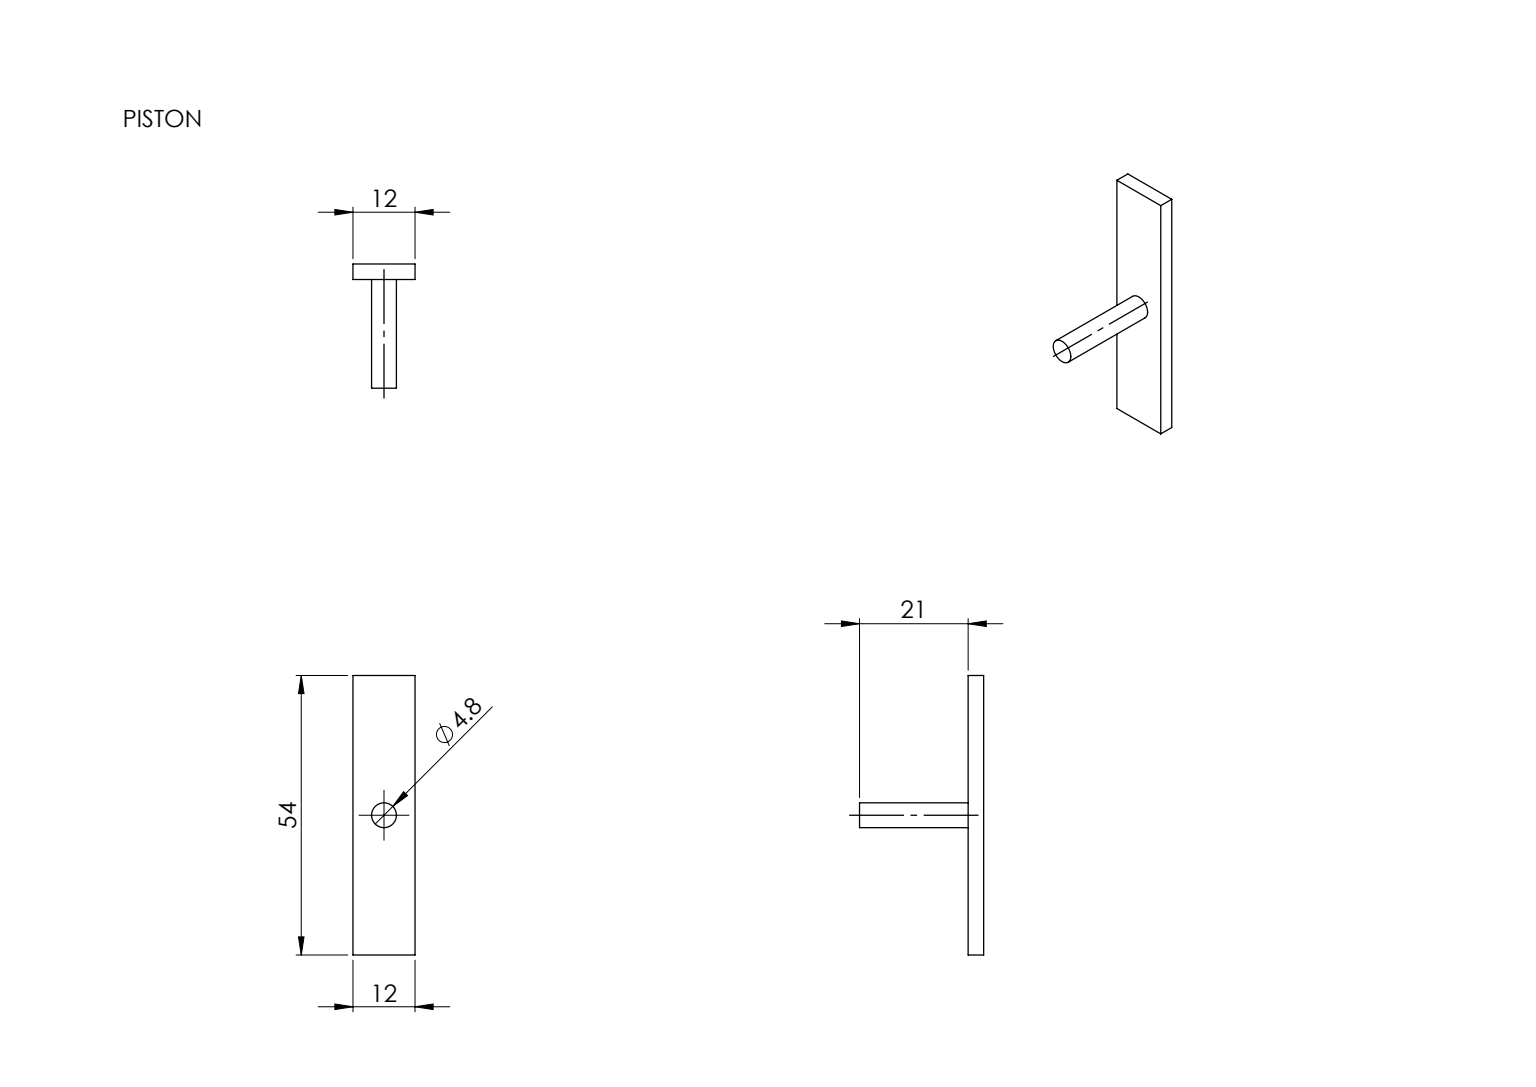
ISO-10303-21;
HEADER;
FILE_DESCRIPTION (('STEP AP214'),
    '1' );
FILE_NAME ('piston.step',
    '2026-10-03T18:28:46',
    ( '' ),
    ( '' ),
    'SwSTEP 2.0',
    'SolidWorks 2026',
    '' );
FILE_SCHEMA (( 'AUTOMOTIVE_DESIGN' ));
ENDSEC;

DATA;
#3=DIRECTION ( 'NONE',  ( -1.000000000000000000, 0.000000000000000000, 0.000000000000000000 ) ) ;
#13=SHAPE_REPRESENTATION ( 'piston', ( #2101 ), #6502 ) ;
#16=PRODUCT_CONTEXT ( 'NONE', #527, 'mechanical' ) ;
#52=ORIENTED_EDGE ( 'NONE', *, *, #338, .F. ) ;
#110=CARTESIAN_POINT ( 'NONE',  ( 5.999999999999999112, -27.00000000000000711, -14.00000000000000178 ) ) ;
#132=LINE ( 'NONE', #5884, #6142 ) ;
#157=CARTESIAN_POINT ( 'NONE',  ( 0.000000000000000000, 0.000000000000000000, 6.999999999999999112 ) ) ;
#184=DIRECTION ( 'NONE',  ( -0.000000000000000000, -0.000000000000000000, -1.000000000000000000 ) ) ;
#232=LINE ( 'NONE', #7430, #6006 ) ;
#246=LINE ( 'NONE', #6800, #847 ) ;
#249=DIRECTION ( 'NONE',  ( -1.000000000000000000, 0.000000000000000000, 0.000000000000000000 ) ) ;
#338=EDGE_CURVE ( 'NONE', #7188, #9680, #5880, .T. ) ;
#349=DIRECTION ( 'NONE',  ( -0.000000000000000000, -1.000000000000000000, -0.000000000000000000 ) ) ;
#383=DIRECTION ( 'NONE',  ( 0.000000000000000000, 0.000000000000000000, 1.000000000000000000 ) ) ;
#496=PRODUCT_DEFINITION ( 'UNKNOWN', '', #10431, #818 ) ;
#527=APPLICATION_CONTEXT ( 'automotive_design' ) ;
#544=ORIENTED_EDGE ( 'NONE', *, *, #10139, .T. ) ;
#558=AXIS2_PLACEMENT_3D ( 'NONE', #2527, #5797, #5015 ) ;
#728=SURFACE_STYLE_USAGE ( .BOTH. , #9540 ) ;
#770=ORIENTED_EDGE ( 'NONE', *, *, #4732, .T. ) ;
#776=ORIENTED_EDGE ( 'NONE', *, *, #9858, .T. ) ;
#779=ORIENTED_EDGE ( 'NONE', *, *, #1512, .F. ) ;
#800=CARTESIAN_POINT ( 'NONE',  ( 2.399999999999999911, 2.939152317953647106E-16, 6.999999999999999112 ) ) ;
#818=PRODUCT_DEFINITION_CONTEXT ( 'detailed design', #5599, 'design' ) ;
#847=VECTOR ( 'NONE', #349, 1000.000000000000000 ) ;
#850=FACE_OUTER_BOUND ( 'NONE', #7920, .T. ) ;
#852=FACE_OUTER_BOUND ( 'NONE', #4523, .T. ) ;
#862=DIRECTION ( 'NONE',  ( 1.000000000000000000, 0.000000000000000000, 0.000000000000000000 ) ) ;
#932=AXIS2_PLACEMENT_3D ( 'NONE', #1647, #10350, #3 ) ;
#956=LINE ( 'NONE', #800, #10182 ) ;
#982=PRESENTATION_STYLE_ASSIGNMENT (( #8411 ) ) ;
#1012=CARTESIAN_POINT ( 'NONE',  ( 0.000000000000000000, 0.000000000000000000, 6.999999999999999112 ) ) ;
#1038=FILL_AREA_STYLE ('',( #3422 ) ) ;
#1126=DIRECTION ( 'NONE',  ( -0.000000000000000000, -0.000000000000000000, -1.000000000000000000 ) ) ;
#1159=DIRECTION ( 'NONE',  ( 0.000000000000000000, 1.000000000000000000, 0.000000000000000000 ) ) ;
#1267=CARTESIAN_POINT ( 'NONE',  ( 5.999999999999999112, 26.99999999999999289, -14.00000000000000178 ) ) ;
#1289=CARTESIAN_POINT ( 'NONE',  ( 5.999999999999999112, 26.99999999999999289, -17.00000000000000000 ) ) ;
#1300=LINE ( 'NONE', #5952, #9319 ) ;
#1316=DIRECTION ( 'NONE',  ( -0.000000000000000000, -0.000000000000000000, -1.000000000000000000 ) ) ;
#1319=CARTESIAN_POINT ( 'NONE',  ( 5.999999999999999112, 26.99999999999999289, -14.00000000000000178 ) ) ;
#1475=CARTESIAN_POINT ( 'NONE',  ( -5.999999999999999112, -27.00000000000000711, -14.00000000000000178 ) ) ;
#1483=ORIENTED_EDGE ( 'NONE', *, *, #8967, .F. ) ;
#1486=ADVANCED_FACE ( 'NONE', ( #5139 ), #9931, .T. ) ;
#1512=EDGE_CURVE ( 'NONE', #9680, #4528, #7119, .T. ) ;
#1647=CARTESIAN_POINT ( 'NONE',  ( 0.000000000000000000, 0.000000000000000000, 6.999999999999999112 ) ) ;
#1677=CARTESIAN_POINT ( 'NONE',  ( 0.000000000000000000, 0.000000000000000000, -14.00000000000000178 ) ) ;
#1697=VERTEX_POINT ( 'NONE', #1319 ) ;
#1711=LINE ( 'NONE', #1866, #9206 ) ;
#1794=EDGE_LOOP ( 'NONE', ( #779, #4050 ) ) ;
#1812=DIRECTION ( 'NONE',  ( 0.000000000000000000, 0.000000000000000000, 1.000000000000000000 ) ) ;
#1814=LINE ( 'NONE', #3454, #9036 ) ;
#1866=CARTESIAN_POINT ( 'NONE',  ( -5.999999999999999112, 26.99999999999999289, -14.00000000000000178 ) ) ;
#1945=DIRECTION ( 'NONE',  ( 0.000000000000000000, 1.000000000000000000, -0.000000000000000000 ) ) ;
#1968=AXIS2_PLACEMENT_3D ( 'NONE', #4462, #8603, #7710 ) ;
#2042=SURFACE_SIDE_STYLE ('',( #6743 ) ) ;
#2050=PLANE ( 'NONE',  #6514 ) ;
#2063=ORIENTED_EDGE ( 'NONE', *, *, #9661, .F. ) ;
#2101=AXIS2_PLACEMENT_3D ( 'NONE', #7090, #5610, #4547 ) ;
#2278=EDGE_CURVE ( 'NONE', #7564, #10476, #6459, .T. ) ;
#2305=EDGE_CURVE ( 'NONE', #8379, #4528, #956, .T. ) ;
#2325=FACE_OUTER_BOUND ( 'NONE', #3648, .T. ) ;
#2338=ADVANCED_FACE ( 'NONE', ( #850 ), #4028, .F. ) ;
#2527=CARTESIAN_POINT ( 'NONE',  ( 0.000000000000000000, 0.000000000000000000, 6.999999999999999112 ) ) ;
#2583=ORIENTED_EDGE ( 'NONE', *, *, #3437, .T. ) ;
#2597=VECTOR ( 'NONE', #4595, 1000.000000000000000 ) ;
#2620=VECTOR ( 'NONE', #1316, 1000.000000000000000 ) ;
#2680=FACE_OUTER_BOUND ( 'NONE', #7404, .T. ) ;
#2743=ORIENTED_EDGE ( 'NONE', *, *, #3577, .T. ) ;
#2758=ORIENTED_EDGE ( 'NONE', *, *, #9103, .F. ) ;
#2818=AXIS2_PLACEMENT_3D ( 'NONE', #6404, #8911, #6513 ) ;
#2874=ORIENTED_EDGE ( 'NONE', *, *, #9103, .T. ) ;
#2957=SHAPE_REPRESENTATION_RELATIONSHIP ( 'NONE' , 'NONE' ,  #13, #2960 ) ;
#2960=ADVANCED_BREP_SHAPE_REPRESENTATION ( '', ( #4712, #2101 ), #6502 ) ;
#2964=DIRECTION ( 'NONE',  ( 0.000000000000000000, 0.000000000000000000, -1.000000000000000000 ) ) ;
#2976=CARTESIAN_POINT ( 'NONE',  ( -2.399999999999999911, 0.000000000000000000, 6.999999999999999112 ) ) ;
#3047=( GEOMETRIC_REPRESENTATION_CONTEXT ( 3 ) GLOBAL_UNCERTAINTY_ASSIGNED_CONTEXT ( ( #6318 ) ) GLOBAL_UNIT_ASSIGNED_CONTEXT ( ( #3624, #9954, #10058 ) ) REPRESENTATION_CONTEXT ( 'NONE', 'WORKASPACE' ) );
#3049=VERTEX_POINT ( 'NONE', #1289 ) ;
#3068=ADVANCED_FACE ( 'NONE', ( #3618 ), #6847, .F. ) ;
#3069=PLANE ( 'NONE',  #10326 ) ;
#3098=VECTOR ( 'NONE', #1159, 1000.000000000000000 ) ;
#3214=ORIENTED_EDGE ( 'NONE', *, *, #8056, .T. ) ;
#3218=AXIS2_PLACEMENT_3D ( 'NONE', #1677, #8203, #6490 ) ;
#3337=DIRECTION ( 'NONE',  ( 1.000000000000000000, -0.000000000000000000, -0.000000000000000000 ) ) ;
#3366=FACE_BOUND ( 'NONE', #1794, .T. ) ;
#3383=ORIENTED_EDGE ( 'NONE', *, *, #9858, .F. ) ;
#3422=FILL_AREA_STYLE_COLOUR ( '', #7101 ) ;
#3437=EDGE_CURVE ( 'NONE', #5860, #7564, #232, .T. ) ;
#3441=DIRECTION ( 'NONE',  ( 0.000000000000000000, 0.000000000000000000, 1.000000000000000000 ) ) ;
#3454=CARTESIAN_POINT ( 'NONE',  ( 5.999999999999999112, -27.00000000000000711, -17.00000000000000000 ) ) ;
#3501=ORIENTED_EDGE ( 'NONE', *, *, #10055, .T. ) ;
#3577=EDGE_CURVE ( 'NONE', #4528, #9680, #4318, .T. ) ;
#3592=( NAMED_UNIT ( * ) SI_UNIT ( $, .STERADIAN. ) SOLID_ANGLE_UNIT ( ) );
#3618=FACE_OUTER_BOUND ( 'NONE', #8196, .T. ) ;
#3624=( LENGTH_UNIT ( ) NAMED_UNIT ( * ) SI_UNIT ( .MILLI., .METRE. ) );
#3648=EDGE_LOOP ( 'NONE', ( #2583, #3383, #4167, #544 ) ) ;
#3662=CARTESIAN_POINT ( 'NONE',  ( 0.000000000000000000, 0.000000000000000000, -14.00000000000000178 ) ) ;
#3724=CARTESIAN_POINT ( 'NONE',  ( -5.999999999999999112, 26.99999999999999289, -14.00000000000000178 ) ) ;
#3725=ORIENTED_EDGE ( 'NONE', *, *, #5954, .T. ) ;
#3745=PRESENTATION_STYLE_ASSIGNMENT (( #728 ) ) ;
#3851=SURFACE_STYLE_FILL_AREA ( #6975 ) ;
#3863=CYLINDRICAL_SURFACE ( 'NONE', #932, 2.399999999999999911 ) ;
#3877=FACE_OUTER_BOUND ( 'NONE', #4533, .T. ) ;
#3891=ADVANCED_FACE ( 'NONE', ( #852 ), #4030, .F. ) ;
#3960=( NAMED_UNIT ( * ) PLANE_ANGLE_UNIT ( ) SI_UNIT ( $, .RADIAN. ) );
#3974=STYLED_ITEM ( 'NONE', ( #3745 ), #2960 ) ;
#4028=PLANE ( 'NONE',  #8996 ) ;
#4030=PLANE ( 'NONE',  #2818 ) ;
#4050=ORIENTED_EDGE ( 'NONE', *, *, #3577, .F. ) ;
#4081=CARTESIAN_POINT ( 'NONE',  ( 5.999999999999999112, 26.99999999999999289, -14.00000000000000178 ) ) ;
#4167=ORIENTED_EDGE ( 'NONE', *, *, #4732, .F. ) ;
#4242=DIRECTION ( 'NONE',  ( 0.000000000000000000, 1.000000000000000000, 0.000000000000000000 ) ) ;
#4291=ADVANCED_FACE ( 'NONE', ( #2325 ), #3069, .F. ) ;
#4292=DIRECTION ( 'NONE',  ( -0.000000000000000000, -0.000000000000000000, -1.000000000000000000 ) ) ;
#4304=MECHANICAL_DESIGN_GEOMETRIC_PRESENTATION_REPRESENTATION('',(#3974),#7361);
#4318=CIRCLE ( 'NONE', #5674, 2.399999999999999911 ) ;
#4340=DIRECTION ( 'NONE',  ( 1.000000000000000000, 0.000000000000000000, 0.000000000000000000 ) ) ;
#4385=CLOSED_SHELL ( 'NONE', ( #5658, #3891, #2338, #4291, #6602, #4600, #3068, #1486, #9647 ) ) ;
#4391=CARTESIAN_POINT ( 'NONE',  ( 0.000000000000000000, 0.000000000000000000, -14.00000000000000178 ) ) ;
#4462=CARTESIAN_POINT ( 'NONE',  ( 0.000000000000000000, 0.000000000000000000, -17.00000000000000000 ) ) ;
#4523=EDGE_LOOP ( 'NONE', ( #3501, #2758, #1483, #3725 ) ) ;
#4528=VERTEX_POINT ( 'NONE', #7348 ) ;
#4533=EDGE_LOOP ( 'NONE', ( #6599, #5263, #6529, #776 ) ) ;
#4547=DIRECTION ( 'NONE',  ( 1.000000000000000000, 0.000000000000000000, 0.000000000000000000 ) ) ;
#4568=VERTEX_POINT ( 'NONE', #10495 ) ;
#4595=DIRECTION ( 'NONE',  ( -1.000000000000000000, 0.000000000000000000, 0.000000000000000000 ) ) ;
#4600=ADVANCED_FACE ( 'NONE', ( #3366, #9047 ), #4957, .T. ) ;
#4705=FACE_OUTER_BOUND ( 'NONE', #5856, .T. ) ;
#4712=MANIFOLD_SOLID_BREP ( 'Boss-Extrude2', #4385 ) ;
#4732=EDGE_CURVE ( 'NONE', #8579, #4568, #246, .T. ) ;
#4746=AXIS2_PLACEMENT_3D ( 'NONE', #4391, #1812, #4340 ) ;
#4767=ORIENTED_EDGE ( 'NONE', *, *, #8967, .T. ) ;
#4821=DIRECTION ( 'NONE',  ( 0.000000000000000000, -0.000000000000000000, -1.000000000000000000 ) ) ;
#4882=DIRECTION ( 'NONE',  ( 0.000000000000000000, 0.000000000000000000, 1.000000000000000000 ) ) ;
#4924=AXIS2_PLACEMENT_3D ( 'NONE', #5873, #5824, #8339 ) ;
#4957=PLANE ( 'NONE',  #3218 ) ;
#5015=DIRECTION ( 'NONE',  ( 1.000000000000000000, 0.000000000000000000, -0.000000000000000000 ) ) ;
#5029=DIRECTION ( 'NONE',  ( -0.000000000000000000, -0.000000000000000000, -1.000000000000000000 ) ) ;
#5078=CARTESIAN_POINT ( 'NONE',  ( -5.999999999999999112, 26.99999999999999289, -17.00000000000000000 ) ) ;
#5119=ORIENTED_EDGE ( 'NONE', *, *, #10139, .F. ) ;
#5139=FACE_OUTER_BOUND ( 'NONE', #9744, .T. ) ;
#5167=ORIENTED_EDGE ( 'NONE', *, *, #338, .T. ) ;
#5230=FILL_AREA_STYLE_COLOUR ( '', #8549 ) ;
#5232=ORIENTED_EDGE ( 'NONE', *, *, #2305, .T. ) ;
#5263=ORIENTED_EDGE ( 'NONE', *, *, #5954, .F. ) ;
#5406=MECHANICAL_DESIGN_GEOMETRIC_PRESENTATION_REPRESENTATION('',(#6249),#3047);
#5427=VECTOR ( 'NONE', #3337, 1000.000000000000000 ) ;
#5599=APPLICATION_CONTEXT ( 'automotive_design' ) ;
#5610=DIRECTION ( 'NONE',  ( 0.000000000000000000, 0.000000000000000000, 1.000000000000000000 ) ) ;
#5658=ADVANCED_FACE ( 'NONE', ( #4705 ), #3863, .T. ) ;
#5674=AXIS2_PLACEMENT_3D ( 'NONE', #3662, #383, #10143 ) ;
#5765=CARTESIAN_POINT ( 'NONE',  ( 5.999999999999999112, -27.00000000000000711, -17.00000000000000000 ) ) ;
#5797=DIRECTION ( 'NONE',  ( 0.000000000000000000, 0.000000000000000000, 1.000000000000000000 ) ) ;
#5824=DIRECTION ( 'NONE',  ( -0.000000000000000000, -0.000000000000000000, -1.000000000000000000 ) ) ;
#5850=CARTESIAN_POINT ( 'NONE',  ( 5.999999999999999112, 26.99999999999999289, -17.00000000000000000 ) ) ;
#5856=EDGE_LOOP ( 'NONE', ( #9307, #5232, #2743, #52 ) ) ;
#5860=VERTEX_POINT ( 'NONE', #5078 ) ;
#5870=EDGE_CURVE ( 'NONE', #8379, #7188, #5987, .T. ) ;
#5873=CARTESIAN_POINT ( 'NONE',  ( 0.000000000000000000, 0.000000000000000000, 6.999999999999999112 ) ) ;
#5880=LINE ( 'NONE', #6034, #10471 ) ;
#5884=CARTESIAN_POINT ( 'NONE',  ( -5.999999999999999112, -27.00000000000000711, -14.00000000000000178 ) ) ;
#5897=CARTESIAN_POINT ( 'NONE',  ( -2.399999999999999911, 0.000000000000000000, -14.00000000000000178 ) ) ;
#5916=LINE ( 'NONE', #110, #8219 ) ;
#5950=ORIENTED_EDGE ( 'NONE', *, *, #1512, .T. ) ;
#5951=DIRECTION ( 'NONE',  ( 0.000000000000000000, 0.000000000000000000, 1.000000000000000000 ) ) ;
#5952=CARTESIAN_POINT ( 'NONE',  ( 5.999999999999999112, -27.00000000000000711, -14.00000000000000178 ) ) ;
#5954=EDGE_CURVE ( 'NONE', #9536, #10476, #5916, .T. ) ;
#5987=CIRCLE ( 'NONE', #10085, 2.399999999999999911 ) ;
#6006=VECTOR ( 'NONE', #8185, 1000.000000000000000 ) ;
#6034=CARTESIAN_POINT ( 'NONE',  ( -2.399999999999999911, 0.000000000000000000, 6.999999999999999112 ) ) ;
#6125=( LENGTH_UNIT ( ) NAMED_UNIT ( * ) SI_UNIT ( .MILLI., .METRE. ) );
#6142=VECTOR ( 'NONE', #184, 1000.000000000000000 ) ;
#6233=CARTESIAN_POINT ( 'NONE',  ( 5.999999999999999112, 26.99999999999999289, -14.00000000000000178 ) ) ;
#6249=STYLED_ITEM ( 'NONE', ( #982 ), #4712 ) ;
#6309=CARTESIAN_POINT ( 'NONE',  ( 5.999999999999999112, -27.00000000000000711, -14.00000000000000178 ) ) ;
#6318=UNCERTAINTY_MEASURE_WITH_UNIT (LENGTH_MEASURE( 1.000000000000000082E-05 ), #3624, 'distance_accuracy_value', 'NONE');
#6331=ORIENTED_EDGE ( 'NONE', *, *, #3437, .F. ) ;
#6344=DIRECTION ( 'NONE',  ( 1.000000000000000000, 0.000000000000000000, 0.000000000000000000 ) ) ;
#6347=ORIENTED_EDGE ( 'NONE', *, *, #10055, .F. ) ;
#6404=CARTESIAN_POINT ( 'NONE',  ( 5.999999999999999112, -27.00000000000000711, -14.00000000000000178 ) ) ;
#6459=LINE ( 'NONE', #5765, #5427 ) ;
#6474=PRODUCT_DEFINITION_SHAPE ( 'NONE', 'NONE',  #496 ) ;
#6490=DIRECTION ( 'NONE',  ( 1.000000000000000000, 0.000000000000000000, -0.000000000000000000 ) ) ;
#6502=( GEOMETRIC_REPRESENTATION_CONTEXT ( 3 ) GLOBAL_UNCERTAINTY_ASSIGNED_CONTEXT ( ( #7923 ) ) GLOBAL_UNIT_ASSIGNED_CONTEXT ( ( #6763, #7623, #3592 ) ) REPRESENTATION_CONTEXT ( 'NONE', 'WORKASPACE' ) );
#6509=ORIENTED_EDGE ( 'NONE', *, *, #9021, .T. ) ;
#6513=DIRECTION ( 'NONE',  ( 0.000000000000000000, 0.000000000000000000, 1.000000000000000000 ) ) ;
#6514=AXIS2_PLACEMENT_3D ( 'NONE', #6309, #1945, #5951 ) ;
#6529=ORIENTED_EDGE ( 'NONE', *, *, #8056, .F. ) ;
#6547=PLANE ( 'NONE',  #558 ) ;
#6599=ORIENTED_EDGE ( 'NONE', *, *, #2278, .T. ) ;
#6602=ADVANCED_FACE ( 'NONE', ( #3877 ), #2050, .F. ) ;
#6672=ORIENTED_EDGE ( 'NONE', *, *, #10200, .T. ) ;
#6743=SURFACE_STYLE_FILL_AREA ( #1038 ) ;
#6763=( LENGTH_UNIT ( ) NAMED_UNIT ( * ) SI_UNIT ( .MILLI., .METRE. ) );
#6800=CARTESIAN_POINT ( 'NONE',  ( -5.999999999999999112, -27.00000000000000711, -14.00000000000000178 ) ) ;
#6817=VECTOR ( 'NONE', #249, 1000.000000000000000 ) ;
#6847=PLANE ( 'NONE',  #1968 ) ;
#6975=FILL_AREA_STYLE ('',( #5230 ) ) ;
#6998=CIRCLE ( 'NONE', #9899, 2.399999999999999911 ) ;
#7030=CARTESIAN_POINT ( 'NONE',  ( -5.999999999999999112, -27.00000000000000711, -17.00000000000000000 ) ) ;
#7090=CARTESIAN_POINT ( 'NONE',  ( 0.000000000000000000, 0.000000000000000000, 0.000000000000000000 ) ) ;
#7101=COLOUR_RGB ( '', 0.72549020, 0.75294118, 0.79215686) ;
#7119=CIRCLE ( 'NONE', #4746, 2.399999999999999911 ) ;
#7184=ORIENTED_EDGE ( 'NONE', *, *, #9661, .T. ) ;
#7188=VERTEX_POINT ( 'NONE', #2976 ) ;
#7348=CARTESIAN_POINT ( 'NONE',  ( 2.399999999999999911, 2.939152317953647106E-16, -14.00000000000000178 ) ) ;
#7361=( GEOMETRIC_REPRESENTATION_CONTEXT ( 3 ) GLOBAL_UNCERTAINTY_ASSIGNED_CONTEXT ( ( #10125 ) ) GLOBAL_UNIT_ASSIGNED_CONTEXT ( ( #6125, #3960, #9483 ) ) REPRESENTATION_CONTEXT ( 'NONE', 'WORKASPACE' ) );
#7404=EDGE_LOOP ( 'NONE', ( #6672, #9721 ) ) ;
#7430=CARTESIAN_POINT ( 'NONE',  ( -5.999999999999999112, -27.00000000000000711, -17.00000000000000000 ) ) ;
#7564=VERTEX_POINT ( 'NONE', #7030 ) ;
#7623=( NAMED_UNIT ( * ) PLANE_ANGLE_UNIT ( ) SI_UNIT ( $, .RADIAN. ) );
#7710=DIRECTION ( 'NONE',  ( 1.000000000000000000, 0.000000000000000000, -0.000000000000000000 ) ) ;
#7827=DIRECTION ( 'NONE',  ( 1.000000000000000000, -0.000000000000000000, -0.000000000000000000 ) ) ;
#7838=LINE ( 'NONE', #1267, #2597 ) ;
#7920=EDGE_LOOP ( 'NONE', ( #7184, #5119, #8733, #2874 ) ) ;
#7923=UNCERTAINTY_MEASURE_WITH_UNIT (LENGTH_MEASURE( 1.000000000000000082E-05 ), #6763, 'distance_accuracy_value', 'NONE');
#8025=SHAPE_DEFINITION_REPRESENTATION ( #6474, #13 ) ;
#8056=EDGE_CURVE ( 'NONE', #4568, #9536, #1300, .T. ) ;
#8136=LINE ( 'NONE', #9224, #3098 ) ;
#8185=DIRECTION ( 'NONE',  ( -0.000000000000000000, -1.000000000000000000, -0.000000000000000000 ) ) ;
#8196=EDGE_LOOP ( 'NONE', ( #6347, #9272, #6331, #2063 ) ) ;
#8203=DIRECTION ( 'NONE',  ( 0.000000000000000000, -0.000000000000000000, 1.000000000000000000 ) ) ;
#8212=EDGE_LOOP ( 'NONE', ( #4767, #6509, #770, #3214 ) ) ;
#8219=VECTOR ( 'NONE', #5029, 1000.000000000000000 ) ;
#8339=DIRECTION ( 'NONE',  ( -1.000000000000000000, 0.000000000000000000, 0.000000000000000000 ) ) ;
#8379=VERTEX_POINT ( 'NONE', #8989 ) ;
#8411=SURFACE_STYLE_USAGE ( .BOTH. , #2042 ) ;
#8549=COLOUR_RGB ( '', 0.72549020, 0.75294118, 0.79215686) ;
#8579=VERTEX_POINT ( 'NONE', #3724 ) ;
#8603=DIRECTION ( 'NONE',  ( 0.000000000000000000, -0.000000000000000000, 1.000000000000000000 ) ) ;
#8733=ORIENTED_EDGE ( 'NONE', *, *, #9021, .F. ) ;
#8911=DIRECTION ( 'NONE',  ( -1.000000000000000000, 0.000000000000000000, 0.000000000000000000 ) ) ;
#8938=PRODUCT ( 'piston', 'piston', '', ( #16 ) ) ;
#8957=DIRECTION ( 'NONE',  ( 0.000000000000000000, -1.000000000000000000, 0.000000000000000000 ) ) ;
#8967=EDGE_CURVE ( 'NONE', #9536, #1697, #8136, .T. ) ;
#8989=CARTESIAN_POINT ( 'NONE',  ( 2.399999999999999911, 2.939152317953647106E-16, 6.999999999999999112 ) ) ;
#8996=AXIS2_PLACEMENT_3D ( 'NONE', #4081, #8957, #4821 ) ;
#9021=EDGE_CURVE ( 'NONE', #1697, #8579, #7838, .T. ) ;
#9036=VECTOR ( 'NONE', #4242, 1000.000000000000000 ) ;
#9047=FACE_OUTER_BOUND ( 'NONE', #8212, .T. ) ;
#9103=EDGE_CURVE ( 'NONE', #1697, #3049, #10081, .T. ) ;
#9206=VECTOR ( 'NONE', #4292, 1000.000000000000000 ) ;
#9224=CARTESIAN_POINT ( 'NONE',  ( 5.999999999999999112, -27.00000000000000711, -14.00000000000000178 ) ) ;
#9272=ORIENTED_EDGE ( 'NONE', *, *, #2278, .F. ) ;
#9307=ORIENTED_EDGE ( 'NONE', *, *, #5870, .F. ) ;
#9319=VECTOR ( 'NONE', #7827, 1000.000000000000000 ) ;
#9483=( NAMED_UNIT ( * ) SI_UNIT ( $, .STERADIAN. ) SOLID_ANGLE_UNIT ( ) );
#9536=VERTEX_POINT ( 'NONE', #9550 ) ;
#9540=SURFACE_SIDE_STYLE ('',( #3851 ) ) ;
#9550=CARTESIAN_POINT ( 'NONE',  ( 5.999999999999999112, -27.00000000000000711, -14.00000000000000178 ) ) ;
#9647=ADVANCED_FACE ( 'NONE', ( #2680 ), #6547, .T. ) ;
#9661=EDGE_CURVE ( 'NONE', #3049, #5860, #9857, .T. ) ;
#9662=DIRECTION ( 'NONE',  ( -0.000000000000000000, -0.000000000000000000, -1.000000000000000000 ) ) ;
#9680=VERTEX_POINT ( 'NONE', #5897 ) ;
#9721=ORIENTED_EDGE ( 'NONE', *, *, #5870, .T. ) ;
#9744=EDGE_LOOP ( 'NONE', ( #10496, #10131, #5167, #5950 ) ) ;
#9857=LINE ( 'NONE', #5850, #6817 ) ;
#9858=EDGE_CURVE ( 'NONE', #4568, #7564, #132, .T. ) ;
#9899=AXIS2_PLACEMENT_3D ( 'NONE', #1012, #4882, #862 ) ;
#9921=DIRECTION ( 'NONE',  ( 1.000000000000000000, 0.000000000000000000, 0.000000000000000000 ) ) ;
#9931=CYLINDRICAL_SURFACE ( 'NONE', #4924, 2.399999999999999911 ) ;
#9954=( NAMED_UNIT ( * ) PLANE_ANGLE_UNIT ( ) SI_UNIT ( $, .RADIAN. ) );
#10055=EDGE_CURVE ( 'NONE', #10476, #3049, #1814, .T. ) ;
#10058=( NAMED_UNIT ( * ) SI_UNIT ( $, .STERADIAN. ) SOLID_ANGLE_UNIT ( ) );
#10081=LINE ( 'NONE', #6233, #2620 ) ;
#10085=AXIS2_PLACEMENT_3D ( 'NONE', #157, #3441, #9921 ) ;
#10125=UNCERTAINTY_MEASURE_WITH_UNIT (LENGTH_MEASURE( 1.000000000000000082E-05 ), #6125, 'distance_accuracy_value', 'NONE');
#10131=ORIENTED_EDGE ( 'NONE', *, *, #10200, .F. ) ;
#10139=EDGE_CURVE ( 'NONE', #8579, #5860, #1711, .T. ) ;
#10143=DIRECTION ( 'NONE',  ( 1.000000000000000000, 0.000000000000000000, 0.000000000000000000 ) ) ;
#10182=VECTOR ( 'NONE', #9662, 1000.000000000000000 ) ;
#10200=EDGE_CURVE ( 'NONE', #7188, #8379, #6998, .T. ) ;
#10326=AXIS2_PLACEMENT_3D ( 'NONE', #1475, #6344, #2964 ) ;
#10350=DIRECTION ( 'NONE',  ( -0.000000000000000000, -0.000000000000000000, -1.000000000000000000 ) ) ;
#10431=PRODUCT_DEFINITION_FORMATION_WITH_SPECIFIED_SOURCE ( 'ANY', '', #8938, .NOT_KNOWN. ) ;
#10461=CARTESIAN_POINT ( 'NONE',  ( 5.999999999999999112, -27.00000000000000711, -17.00000000000000000 ) ) ;
#10471=VECTOR ( 'NONE', #1126, 1000.000000000000000 ) ;
#10476=VERTEX_POINT ( 'NONE', #10461 ) ;
#10495=CARTESIAN_POINT ( 'NONE',  ( -5.999999999999999112, -27.00000000000000711, -14.00000000000000178 ) ) ;
#10496=ORIENTED_EDGE ( 'NONE', *, *, #2305, .F. ) ;
ENDSEC;
END-ISO-10303-21;
